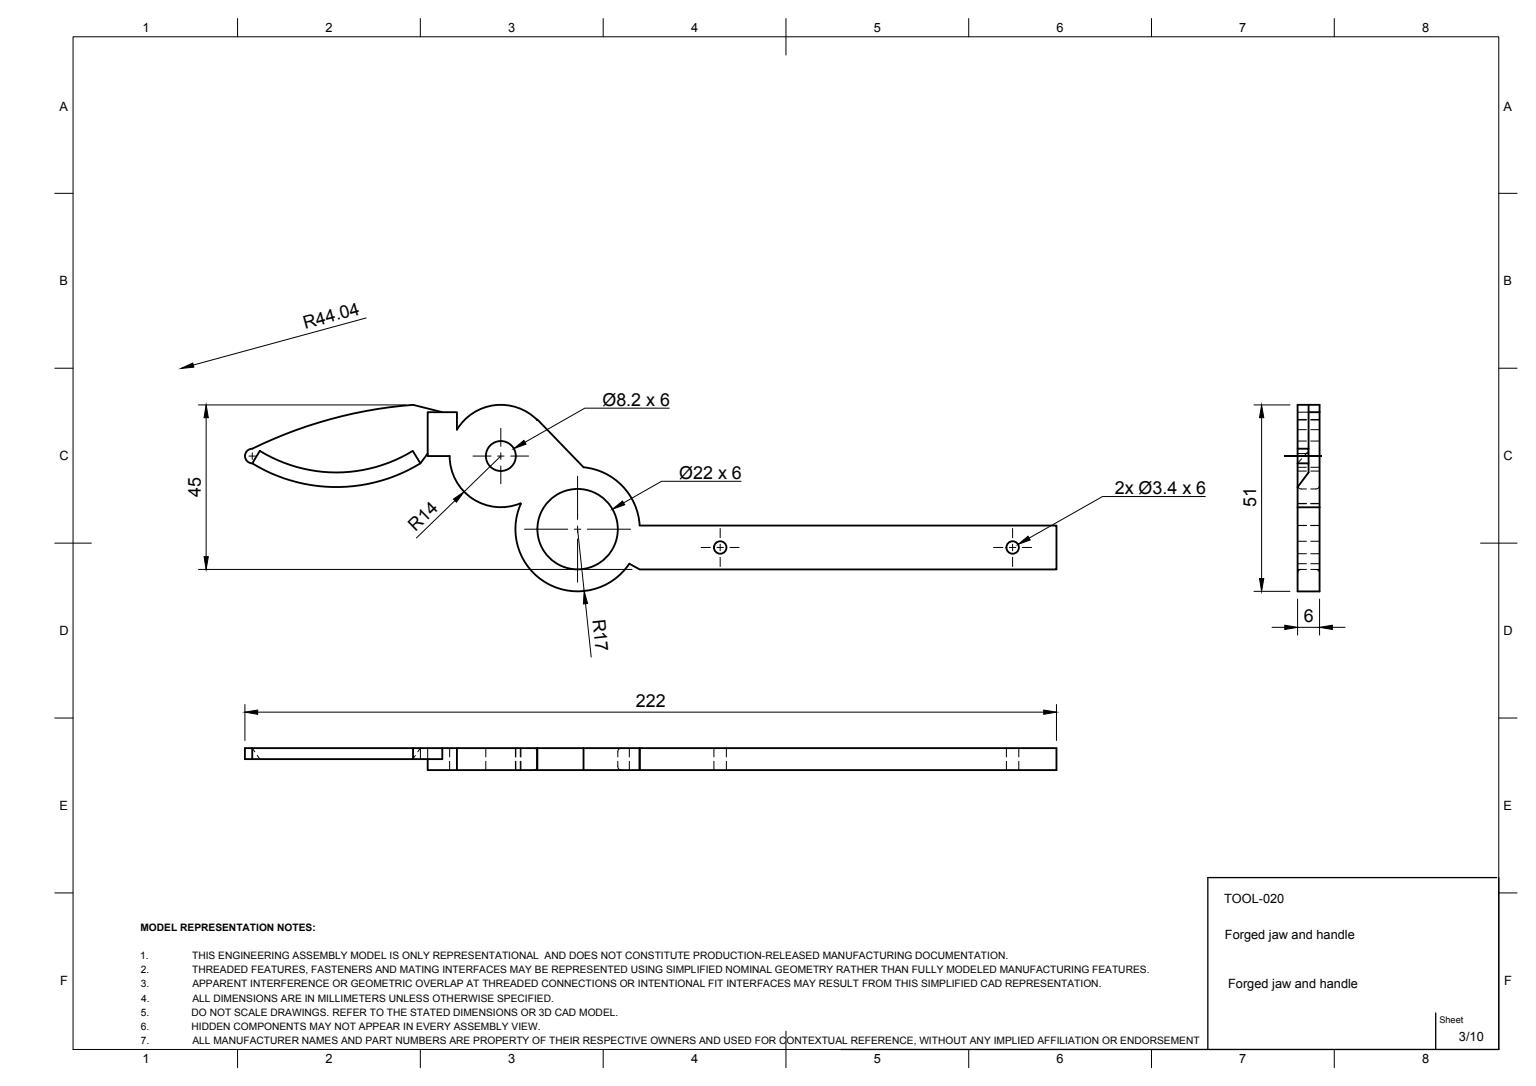
ISO-10303-21;
HEADER;
/* Generated by software containing ST-Developer
 * from STEP Tools, Inc. (www.steptools.com) 
 */

FILE_DESCRIPTION(
/* description */ (''),
/* implementation_level */ '2;1');

FILE_NAME(
/* name */ 'Forged jaw and handle.step',
/* time_stamp */ '2026-11-10T09:09:39-08:00',
/* author */ (''),
/* organization */ (''),
/* preprocessor_version */ 'ST-DEVELOPER v20.2',
/* originating_system */ 'Autodesk Translation Framework v15.17.0.0',
/* authorisation */ '');

FILE_SCHEMA (('AUTOMOTIVE_DESIGN { 1 0 10303 214 3 1 1 }'));
ENDSEC;

DATA;
#10=MECHANICAL_DESIGN_GEOMETRIC_PRESENTATION_REPRESENTATION('',(#555),#18353);
#537=SHAPE_REPRESENTATION_RELATIONSHIP('SRR','None',#18397,#546);
#546=ADVANCED_BREP_SHAPE_REPRESENTATION('',(#564),#18343);
#555=STYLED_ITEM('',(#18456),#564);
#564=MANIFOLD_SOLID_BREP('Body1',#6486);
#573=TOROIDAL_SURFACE('',#6634,1.2,0.1);
#574=TOROIDAL_SURFACE('',#6644,1.2,0.1);
#575=FACE_BOUND('',#1173,.T.);
#576=FACE_BOUND('',#1174,.T.);
#577=FACE_BOUND('',#1175,.T.);
#578=FACE_BOUND('',#1176,.T.);
#579=FACE_BOUND('',#1180,.T.);
#580=FACE_BOUND('',#1181,.T.);
#581=FACE_BOUND('',#1182,.T.);
#582=FACE_BOUND('',#1183,.T.);
#638=CONICAL_SURFACE('',#6607,4.2044765934785,0.927295218001611);
#640=PLANE('',#6606);
#641=PLANE('',#6610);
#642=PLANE('',#6611);
#643=PLANE('',#6612);
#644=PLANE('',#6619);
#645=PLANE('',#6620);
#646=PLANE('',#6621);
#647=PLANE('',#6622);
#648=PLANE('',#6623);
#649=PLANE('',#6630);
#650=PLANE('',#6641);
#651=PLANE('',#6648);
#652=PLANE('',#6649);
#653=PLANE('',#6650);
#654=PLANE('',#6651);
#655=PLANE('',#6652);
#656=PLANE('',#6653);
#657=PLANE('',#6654);
#658=PLANE('',#6655);
#782=FACE_OUTER_BOUND('',#1155,.T.);
#783=FACE_OUTER_BOUND('',#1156,.T.);
#784=FACE_OUTER_BOUND('',#1157,.T.);
#785=FACE_OUTER_BOUND('',#1158,.T.);
#786=FACE_OUTER_BOUND('',#1159,.T.);
#787=FACE_OUTER_BOUND('',#1160,.T.);
#788=FACE_OUTER_BOUND('',#1161,.T.);
#789=FACE_OUTER_BOUND('',#1162,.T.);
#790=FACE_OUTER_BOUND('',#1163,.T.);
#791=FACE_OUTER_BOUND('',#1164,.T.);
#792=FACE_OUTER_BOUND('',#1165,.T.);
#793=FACE_OUTER_BOUND('',#1166,.T.);
#794=FACE_OUTER_BOUND('',#1167,.T.);
#795=FACE_OUTER_BOUND('',#1168,.T.);
#796=FACE_OUTER_BOUND('',#1169,.T.);
#797=FACE_OUTER_BOUND('',#1170,.T.);
#798=FACE_OUTER_BOUND('',#1171,.T.);
#799=FACE_OUTER_BOUND('',#1172,.T.);
#800=FACE_OUTER_BOUND('',#1177,.T.);
#801=FACE_OUTER_BOUND('',#1178,.T.);
#802=FACE_OUTER_BOUND('',#1179,.T.);
#803=FACE_OUTER_BOUND('',#1184,.T.);
#804=FACE_OUTER_BOUND('',#1185,.T.);
#805=FACE_OUTER_BOUND('',#1186,.T.);
#806=FACE_OUTER_BOUND('',#1187,.T.);
#807=FACE_OUTER_BOUND('',#1188,.T.);
#808=FACE_OUTER_BOUND('',#1189,.T.);
#809=FACE_OUTER_BOUND('',#1190,.T.);
#810=FACE_OUTER_BOUND('',#1191,.T.);
#811=FACE_OUTER_BOUND('',#1192,.T.);
#812=FACE_OUTER_BOUND('',#1193,.T.);
#813=FACE_OUTER_BOUND('',#1194,.T.);
#1155=EDGE_LOOP('',(#4108,#4109,#4110,#4111));
#1156=EDGE_LOOP('',(#4112,#4113,#4114,#4115));
#1157=EDGE_LOOP('',(#4116,#4117,#4118,#4119));
#1158=EDGE_LOOP('',(#4120,#4121,#4122));
#1159=EDGE_LOOP('',(#4123,#4124,#4125,#4126));
#1160=EDGE_LOOP('',(#4127,#4128,#4129));
#1161=EDGE_LOOP('',(#4130,#4131,#4132,#4133));
#1162=EDGE_LOOP('',(#4134,#4135,#4136,#4137));
#1163=EDGE_LOOP('',(#4138,#4139,#4140,#4141));
#1164=EDGE_LOOP('',(#4142,#4143,#4144,#4145));
#1165=EDGE_LOOP('',(#4146,#4147,#4148,#4149,#4150,#4151,#4152,#4153,#4154));
#1166=EDGE_LOOP('',(#4155,#4156,#4157,#4158,#4159,#4160));
#1167=EDGE_LOOP('',(#4161,#4162,#4163,#4164,#4165,#4166));
#1168=EDGE_LOOP('',(#4167,#4168,#4169,#4170));
#1169=EDGE_LOOP('',(#4171,#4172,#4173,#4174));
#1170=EDGE_LOOP('',(#4175,#4176,#4177,#4178));
#1171=EDGE_LOOP('',(#4179,#4180,#4181,#4182));
#1172=EDGE_LOOP('',(#4183,#4184,#4185,#4186,#4187,#4188,#4189,#4190,#4191,
#4192,#4193,#4194,#4195,#4196,#4197,#4198));
#1173=EDGE_LOOP('',(#4199));
#1174=EDGE_LOOP('',(#4200));
#1175=EDGE_LOOP('',(#4201));
#1176=EDGE_LOOP('',(#4202));
#1177=EDGE_LOOP('',(#4203,#4204,#4205,#4206));
#1178=EDGE_LOOP('',(#4207,#4208,#4209,#4210,#4211));
#1179=EDGE_LOOP('',(#4212,#4213,#4214,#4215,#4216,#4217,#4218,#4219,#4220,
#4221,#4222,#4223,#4224,#4225,#4226,#4227,#4228,#4229,#4230,#4231,#4232));
#1180=EDGE_LOOP('',(#4233));
#1181=EDGE_LOOP('',(#4234));
#1182=EDGE_LOOP('',(#4235));
#1183=EDGE_LOOP('',(#4236));
#1184=EDGE_LOOP('',(#4237,#4238,#4239,#4240,#4241));
#1185=EDGE_LOOP('',(#4242,#4243,#4244,#4245));
#1186=EDGE_LOOP('',(#4246,#4247,#4248,#4249));
#1187=EDGE_LOOP('',(#4250,#4251,#4252,#4253));
#1188=EDGE_LOOP('',(#4254,#4255,#4256,#4257));
#1189=EDGE_LOOP('',(#4258,#4259,#4260,#4261));
#1190=EDGE_LOOP('',(#4262,#4263,#4264,#4265));
#1191=EDGE_LOOP('',(#4266,#4267,#4268,#4269));
#1192=EDGE_LOOP('',(#4270,#4271,#4272,#4273));
#1193=EDGE_LOOP('',(#4274,#4275,#4276,#4277));
#1194=EDGE_LOOP('',(#4278,#4279,#4280,#4281));
#1591=LINE('',#8466,#1995);
#1592=LINE('',#8472,#1996);
#1593=LINE('',#8478,#1997);
#1594=LINE('',#8483,#1998);
#1595=LINE('',#8485,#1999);
#1596=LINE('',#8486,#2000);
#1597=LINE('',#8490,#2001);
#1598=LINE('',#8495,#2002);
#1599=LINE('',#8496,#2003);
#1600=LINE('',#8500,#2004);
#1601=LINE('',#8501,#2005);
#1602=LINE('',#8502,#2006);
#1603=LINE('',#8506,#2007);
#1604=LINE('',#8508,#2008);
#1605=LINE('',#8510,#2009);
#1606=LINE('',#8511,#2010);
#1607=LINE('',#8517,#2011);
#1608=LINE('',#8523,#2012);
#1609=LINE('',#8524,#2013);
#1610=LINE('',#8527,#2014);
#1611=LINE('',#8529,#2015);
#1612=LINE('',#8531,#2016);
#1613=LINE('',#8532,#2017);
#1614=LINE('',#8535,#2018);
#1615=LINE('',#8537,#2019);
#1616=LINE('',#8538,#2020);
#1617=LINE('',#8542,#2021);
#1618=LINE('',#8543,#2022);
#1619=LINE('',#8544,#2023);
#1620=LINE('',#8548,#2024);
#1621=LINE('',#8549,#2025);
#1622=LINE('',#8550,#2026);
#1623=LINE('',#8555,#2027);
#1624=LINE('',#8561,#2028);
#1625=LINE('',#8565,#2029);
#1626=LINE('',#8569,#2030);
#1627=LINE('',#8571,#2031);
#1628=LINE('',#8573,#2032);
#1629=LINE('',#8575,#2033);
#1630=LINE('',#8577,#2034);
#1631=LINE('',#8581,#2035);
#1632=LINE('',#8582,#2036);
#1633=LINE('',#8596,#2037);
#1634=LINE('',#8599,#2038);
#1635=LINE('',#8601,#2039);
#1636=LINE('',#8605,#2040);
#1637=LINE('',#8607,#2041);
#1638=LINE('',#8609,#2042);
#1639=LINE('',#8611,#2043);
#1640=LINE('',#8613,#2044);
#1641=LINE('',#8616,#2045);
#1642=LINE('',#8620,#2046);
#1643=LINE('',#8621,#2047);
#1644=LINE('',#8623,#2048);
#1645=LINE('',#8624,#2049);
#1646=LINE('',#8626,#2050);
#1647=LINE('',#8628,#2051);
#1648=LINE('',#8631,#2052);
#1649=LINE('',#8634,#2053);
#1650=LINE('',#8636,#2054);
#1995=VECTOR('',#7090,0.17);
#1996=VECTOR('',#7097,0.17);
#1997=VECTOR('',#7104,0.41);
#1998=VECTOR('',#7109,1.);
#1999=VECTOR('',#7110,1.);
#2000=VECTOR('',#7111,1.);
#2001=VECTOR('',#7114,1.);
#2002=VECTOR('',#7121,1.);
#2003=VECTOR('',#7122,1.);
#2004=VECTOR('',#7125,1.);
#2005=VECTOR('',#7126,1.);
#2006=VECTOR('',#7127,1.);
#2007=VECTOR('',#7130,1.);
#2008=VECTOR('',#7131,1.);
#2009=VECTOR('',#7132,1.);
#2010=VECTOR('',#7133,1.);
#2011=VECTOR('',#7140,1.);
#2012=VECTOR('',#7149,1.);
#2013=VECTOR('',#7150,1.);
#2014=VECTOR('',#7153,1.);
#2015=VECTOR('',#7154,1.);
#2016=VECTOR('',#7155,1.);
#2017=VECTOR('',#7156,1.);
#2018=VECTOR('',#7159,1.);
#2019=VECTOR('',#7160,1.);
#2020=VECTOR('',#7161,1.);
#2021=VECTOR('',#7164,1.);
#2022=VECTOR('',#7165,1.);
#2023=VECTOR('',#7166,1.);
#2024=VECTOR('',#7169,1.);
#2025=VECTOR('',#7170,1.);
#2026=VECTOR('',#7171,1.);
#2027=VECTOR('',#7176,1.);
#2028=VECTOR('',#7183,1.);
#2029=VECTOR('',#7188,1.);
#2030=VECTOR('',#7191,1.);
#2031=VECTOR('',#7192,1.);
#2032=VECTOR('',#7193,1.);
#2033=VECTOR('',#7194,1.);
#2034=VECTOR('',#7195,1.);
#2035=VECTOR('',#7198,1.);
#2036=VECTOR('',#7199,1.);
#2037=VECTOR('',#7216,1.1);
#2038=VECTOR('',#7219,1.);
#2039=VECTOR('',#7220,1.);
#2040=VECTOR('',#7223,1.);
#2041=VECTOR('',#7224,1.);
#2042=VECTOR('',#7225,1.);
#2043=VECTOR('',#7226,1.);
#2044=VECTOR('',#7227,1.);
#2045=VECTOR('',#7230,1.);
#2046=VECTOR('',#7237,1.);
#2047=VECTOR('',#7238,1.);
#2048=VECTOR('',#7241,1.);
#2049=VECTOR('',#7242,1.);
#2050=VECTOR('',#7245,1.);
#2051=VECTOR('',#7248,1.);
#2052=VECTOR('',#7253,1.);
#2053=VECTOR('',#7258,1.);
#2054=VECTOR('',#7261,1.);
#2399=CIRCLE('',#6598,0.17);
#2400=CIRCLE('',#6599,0.17);
#2401=CIRCLE('',#6601,0.17);
#2402=CIRCLE('',#6602,0.17);
#2403=CIRCLE('',#6604,0.41);
#2404=CIRCLE('',#6605,0.41);
#2405=CIRCLE('',#6608,4.4044765934785);
#2406=CIRCLE('',#6609,4.0044765934785);
#2407=CIRCLE('',#6614,0.2);
#2408=CIRCLE('',#6615,0.2);
#2409=CIRCLE('',#6617,12.0894198846614);
#2410=CIRCLE('',#6618,12.0894198846614);
#2411=CIRCLE('',#6625,1.4);
#2412=CIRCLE('',#6626,1.4);
#2413=CIRCLE('',#6628,1.4);
#2414=CIRCLE('',#6629,1.4);
#2415=CIRCLE('',#6631,1.7);
#2416=CIRCLE('',#6632,1.7);
#2417=CIRCLE('',#6633,1.2);
#2418=CIRCLE('',#6635,1.2);
#2419=CIRCLE('',#6636,0.1);
#2420=CIRCLE('',#6637,1.1);
#2421=CIRCLE('',#6639,1.1);
#2422=CIRCLE('',#6640,1.1);
#2423=CIRCLE('',#6642,1.7);
#2424=CIRCLE('',#6643,1.7);
#2425=CIRCLE('',#6645,0.1);
#2566=VERTEX_POINT('',#8463);
#2567=VERTEX_POINT('',#8465);
#2568=VERTEX_POINT('',#8469);
#2569=VERTEX_POINT('',#8471);
#2570=VERTEX_POINT('',#8475);
#2571=VERTEX_POINT('',#8477);
#2572=VERTEX_POINT('',#8481);
#2573=VERTEX_POINT('',#8482);
#2574=VERTEX_POINT('',#8484);
#2575=VERTEX_POINT('',#8488);
#2576=VERTEX_POINT('',#8489);
#2577=VERTEX_POINT('',#8494);
#2578=VERTEX_POINT('',#8498);
#2579=VERTEX_POINT('',#8499);
#2580=VERTEX_POINT('',#8504);
#2581=VERTEX_POINT('',#8505);
#2582=VERTEX_POINT('',#8507);
#2583=VERTEX_POINT('',#8509);
#2584=VERTEX_POINT('',#8513);
#2585=VERTEX_POINT('',#8515);
#2586=VERTEX_POINT('',#8522);
#2587=VERTEX_POINT('',#8526);
#2588=VERTEX_POINT('',#8528);
#2589=VERTEX_POINT('',#8530);
#2590=VERTEX_POINT('',#8534);
#2591=VERTEX_POINT('',#8536);
#2592=VERTEX_POINT('',#8540);
#2593=VERTEX_POINT('',#8541);
#2594=VERTEX_POINT('',#8546);
#2595=VERTEX_POINT('',#8547);
#2596=VERTEX_POINT('',#8552);
#2597=VERTEX_POINT('',#8554);
#2598=VERTEX_POINT('',#8558);
#2599=VERTEX_POINT('',#8560);
#2600=VERTEX_POINT('',#8564);
#2601=VERTEX_POINT('',#8566);
#2602=VERTEX_POINT('',#8568);
#2603=VERTEX_POINT('',#8570);
#2604=VERTEX_POINT('',#8572);
#2605=VERTEX_POINT('',#8574);
#2606=VERTEX_POINT('',#8576);
#2607=VERTEX_POINT('',#8578);
#2608=VERTEX_POINT('',#8580);
#2609=VERTEX_POINT('',#8583);
#2610=VERTEX_POINT('',#8586);
#2611=VERTEX_POINT('',#8588);
#2612=VERTEX_POINT('',#8592);
#2613=VERTEX_POINT('',#8593);
#2614=VERTEX_POINT('',#8598);
#2615=VERTEX_POINT('',#8600);
#2616=VERTEX_POINT('',#8602);
#2617=VERTEX_POINT('',#8604);
#2618=VERTEX_POINT('',#8606);
#2619=VERTEX_POINT('',#8608);
#2620=VERTEX_POINT('',#8610);
#2621=VERTEX_POINT('',#8612);
#2622=VERTEX_POINT('',#8614);
#3171=EDGE_CURVE('',#2566,#2566,#2399,.T.);
#3172=EDGE_CURVE('',#2566,#2567,#1591,.T.);
#3173=EDGE_CURVE('',#2567,#2567,#2400,.T.);
#3174=EDGE_CURVE('',#2568,#2568,#2401,.T.);
#3175=EDGE_CURVE('',#2568,#2569,#1592,.T.);
#3176=EDGE_CURVE('',#2569,#2569,#2402,.T.);
#3177=EDGE_CURVE('',#2570,#2570,#2403,.T.);
#3178=EDGE_CURVE('',#2570,#2571,#1593,.T.);
#3179=EDGE_CURVE('',#2571,#2571,#2404,.T.);
#3180=EDGE_CURVE('',#2572,#2573,#1594,.T.);
#3181=EDGE_CURVE('',#2574,#2572,#1595,.T.);
#3182=EDGE_CURVE('',#2574,#2573,#1596,.T.);
#3183=EDGE_CURVE('',#2575,#2576,#1597,.T.);
#3184=EDGE_CURVE('',#2575,#2574,#2405,.T.);
#3185=EDGE_CURVE('',#2576,#2572,#2406,.T.);
#3186=EDGE_CURVE('',#2577,#2576,#1598,.T.);
#3187=EDGE_CURVE('',#2575,#2577,#1599,.T.);
#3188=EDGE_CURVE('',#2578,#2579,#1600,.T.);
#3189=EDGE_CURVE('',#2573,#2578,#1601,.T.);
#3190=EDGE_CURVE('',#2579,#2574,#1602,.T.);
#3191=EDGE_CURVE('',#2580,#2581,#1603,.T.);
#3192=EDGE_CURVE('',#2580,#2582,#1604,.T.);
#3193=EDGE_CURVE('',#2583,#2582,#1605,.T.);
#3194=EDGE_CURVE('',#2581,#2583,#1606,.T.);
#3195=EDGE_CURVE('',#2584,#2575,#2407,.T.);
#3196=EDGE_CURVE('',#2585,#2577,#2408,.T.);
#3197=EDGE_CURVE('',#2584,#2585,#1607,.T.);
#3198=EDGE_CURVE('',#2580,#2584,#2409,.T.);
#3199=EDGE_CURVE('',#2582,#2585,#2410,.T.);
#3200=EDGE_CURVE('',#2586,#2578,#1608,.T.);
#3201=EDGE_CURVE('',#2583,#2586,#1609,.T.);
#3202=EDGE_CURVE('',#2586,#2587,#1610,.T.);
#3203=EDGE_CURVE('',#2588,#2587,#1611,.T.);
#3204=EDGE_CURVE('',#2589,#2588,#1612,.T.);
#3205=EDGE_CURVE('',#2581,#2589,#1613,.T.);
#3206=EDGE_CURVE('',#2590,#2579,#1614,.T.);
#3207=EDGE_CURVE('',#2590,#2591,#1615,.T.);
#3208=EDGE_CURVE('',#2587,#2591,#1616,.T.);
#3209=EDGE_CURVE('',#2592,#2593,#1617,.T.);
#3210=EDGE_CURVE('',#2591,#2592,#1618,.T.);
#3211=EDGE_CURVE('',#2593,#2590,#1619,.T.);
#3212=EDGE_CURVE('',#2594,#2595,#1620,.T.);
#3213=EDGE_CURVE('',#2589,#2594,#1621,.T.);
#3214=EDGE_CURVE('',#2595,#2588,#1622,.T.);
#3215=EDGE_CURVE('',#2593,#2596,#2411,.T.);
#3216=EDGE_CURVE('',#2596,#2597,#1623,.T.);
#3217=EDGE_CURVE('',#2592,#2597,#2412,.T.);
#3218=EDGE_CURVE('',#2598,#2595,#2413,.T.);
#3219=EDGE_CURVE('',#2598,#2599,#1624,.T.);
#3220=EDGE_CURVE('',#2599,#2594,#2414,.T.);
#3221=EDGE_CURVE('',#2597,#2600,#1625,.T.);
#3222=EDGE_CURVE('',#2600,#2601,#2415,.T.);
#3223=EDGE_CURVE('',#2601,#2602,#1626,.T.);
#3224=EDGE_CURVE('',#2602,#2603,#1627,.T.);
#3225=EDGE_CURVE('',#2603,#2604,#1628,.T.);
#3226=EDGE_CURVE('',#2604,#2605,#1629,.T.);
#3227=EDGE_CURVE('',#2605,#2606,#1630,.T.);
#3228=EDGE_CURVE('',#2606,#2607,#2416,.T.);
#3229=EDGE_CURVE('',#2607,#2608,#1631,.T.);
#3230=EDGE_CURVE('',#2608,#2598,#1632,.T.);
#3231=EDGE_CURVE('',#2609,#2609,#2417,.T.);
#3232=EDGE_CURVE('',#2610,#2610,#2418,.T.);
#3233=EDGE_CURVE('',#2610,#2611,#2419,.T.);
#3234=EDGE_CURVE('',#2611,#2611,#2420,.T.);
#3235=EDGE_CURVE('',#2612,#2613,#2421,.T.);
#3236=EDGE_CURVE('',#2613,#2612,#2422,.T.);
#3237=EDGE_CURVE('',#2613,#2611,#1633,.T.);
#3238=EDGE_CURVE('',#2614,#2599,#1634,.T.);
#3239=EDGE_CURVE('',#2615,#2614,#1635,.T.);
#3240=EDGE_CURVE('',#2616,#2615,#2423,.T.);
#3241=EDGE_CURVE('',#2617,#2616,#1636,.T.);
#3242=EDGE_CURVE('',#2618,#2617,#1637,.T.);
#3243=EDGE_CURVE('',#2619,#2618,#1638,.T.);
#3244=EDGE_CURVE('',#2620,#2619,#1639,.T.);
#3245=EDGE_CURVE('',#2621,#2620,#1640,.T.);
#3246=EDGE_CURVE('',#2622,#2621,#2424,.T.);
#3247=EDGE_CURVE('',#2596,#2622,#1641,.T.);
#3248=EDGE_CURVE('',#2609,#2612,#2425,.T.);
#3249=EDGE_CURVE('',#2607,#2615,#1642,.T.);
#3250=EDGE_CURVE('',#2616,#2606,#1643,.T.);
#3251=EDGE_CURVE('',#2622,#2600,#1644,.T.);
#3252=EDGE_CURVE('',#2601,#2621,#1645,.T.);
#3253=EDGE_CURVE('',#2620,#2602,#1646,.T.);
#3254=EDGE_CURVE('',#2617,#2605,#1647,.T.);
#3255=EDGE_CURVE('',#2614,#2608,#1648,.T.);
#3256=EDGE_CURVE('',#2618,#2604,#1649,.T.);
#3257=EDGE_CURVE('',#2619,#2603,#1650,.T.);
#4108=ORIENTED_EDGE('',*,*,#3171,.F.);
#4109=ORIENTED_EDGE('',*,*,#3172,.T.);
#4110=ORIENTED_EDGE('',*,*,#3173,.F.);
#4111=ORIENTED_EDGE('',*,*,#3172,.F.);
#4112=ORIENTED_EDGE('',*,*,#3174,.F.);
#4113=ORIENTED_EDGE('',*,*,#3175,.T.);
#4114=ORIENTED_EDGE('',*,*,#3176,.F.);
#4115=ORIENTED_EDGE('',*,*,#3175,.F.);
#4116=ORIENTED_EDGE('',*,*,#3177,.F.);
#4117=ORIENTED_EDGE('',*,*,#3178,.T.);
#4118=ORIENTED_EDGE('',*,*,#3179,.F.);
#4119=ORIENTED_EDGE('',*,*,#3178,.F.);
#4120=ORIENTED_EDGE('',*,*,#3180,.F.);
#4121=ORIENTED_EDGE('',*,*,#3181,.F.);
#4122=ORIENTED_EDGE('',*,*,#3182,.T.);
#4123=ORIENTED_EDGE('',*,*,#3183,.F.);
#4124=ORIENTED_EDGE('',*,*,#3184,.T.);
#4125=ORIENTED_EDGE('',*,*,#3181,.T.);
#4126=ORIENTED_EDGE('',*,*,#3185,.F.);
#4127=ORIENTED_EDGE('',*,*,#3186,.F.);
#4128=ORIENTED_EDGE('',*,*,#3187,.F.);
#4129=ORIENTED_EDGE('',*,*,#3183,.T.);
#4130=ORIENTED_EDGE('',*,*,#3188,.F.);
#4131=ORIENTED_EDGE('',*,*,#3189,.F.);
#4132=ORIENTED_EDGE('',*,*,#3182,.F.);
#4133=ORIENTED_EDGE('',*,*,#3190,.F.);
#4134=ORIENTED_EDGE('',*,*,#3191,.F.);
#4135=ORIENTED_EDGE('',*,*,#3192,.T.);
#4136=ORIENTED_EDGE('',*,*,#3193,.F.);
#4137=ORIENTED_EDGE('',*,*,#3194,.F.);
#4138=ORIENTED_EDGE('',*,*,#3195,.T.);
#4139=ORIENTED_EDGE('',*,*,#3187,.T.);
#4140=ORIENTED_EDGE('',*,*,#3196,.F.);
#4141=ORIENTED_EDGE('',*,*,#3197,.F.);
#4142=ORIENTED_EDGE('',*,*,#3198,.T.);
#4143=ORIENTED_EDGE('',*,*,#3197,.T.);
#4144=ORIENTED_EDGE('',*,*,#3199,.F.);
#4145=ORIENTED_EDGE('',*,*,#3192,.F.);
#4146=ORIENTED_EDGE('',*,*,#3180,.T.);
#4147=ORIENTED_EDGE('',*,*,#3189,.T.);
#4148=ORIENTED_EDGE('',*,*,#3200,.F.);
#4149=ORIENTED_EDGE('',*,*,#3201,.F.);
#4150=ORIENTED_EDGE('',*,*,#3193,.T.);
#4151=ORIENTED_EDGE('',*,*,#3199,.T.);
#4152=ORIENTED_EDGE('',*,*,#3196,.T.);
#4153=ORIENTED_EDGE('',*,*,#3186,.T.);
#4154=ORIENTED_EDGE('',*,*,#3185,.T.);
#4155=ORIENTED_EDGE('',*,*,#3194,.T.);
#4156=ORIENTED_EDGE('',*,*,#3201,.T.);
#4157=ORIENTED_EDGE('',*,*,#3202,.T.);
#4158=ORIENTED_EDGE('',*,*,#3203,.F.);
#4159=ORIENTED_EDGE('',*,*,#3204,.F.);
#4160=ORIENTED_EDGE('',*,*,#3205,.F.);
#4161=ORIENTED_EDGE('',*,*,#3200,.T.);
#4162=ORIENTED_EDGE('',*,*,#3188,.T.);
#4163=ORIENTED_EDGE('',*,*,#3206,.F.);
#4164=ORIENTED_EDGE('',*,*,#3207,.T.);
#4165=ORIENTED_EDGE('',*,*,#3208,.F.);
#4166=ORIENTED_EDGE('',*,*,#3202,.F.);
#4167=ORIENTED_EDGE('',*,*,#3209,.F.);
#4168=ORIENTED_EDGE('',*,*,#3210,.F.);
#4169=ORIENTED_EDGE('',*,*,#3207,.F.);
#4170=ORIENTED_EDGE('',*,*,#3211,.F.);
#4171=ORIENTED_EDGE('',*,*,#3212,.F.);
#4172=ORIENTED_EDGE('',*,*,#3213,.F.);
#4173=ORIENTED_EDGE('',*,*,#3204,.T.);
#4174=ORIENTED_EDGE('',*,*,#3214,.F.);
#4175=ORIENTED_EDGE('',*,*,#3209,.T.);
#4176=ORIENTED_EDGE('',*,*,#3215,.T.);
#4177=ORIENTED_EDGE('',*,*,#3216,.T.);
#4178=ORIENTED_EDGE('',*,*,#3217,.F.);
#4179=ORIENTED_EDGE('',*,*,#3212,.T.);
#4180=ORIENTED_EDGE('',*,*,#3218,.F.);
#4181=ORIENTED_EDGE('',*,*,#3219,.T.);
#4182=ORIENTED_EDGE('',*,*,#3220,.T.);
#4183=ORIENTED_EDGE('',*,*,#3217,.T.);
#4184=ORIENTED_EDGE('',*,*,#3221,.T.);
#4185=ORIENTED_EDGE('',*,*,#3222,.T.);
#4186=ORIENTED_EDGE('',*,*,#3223,.T.);
#4187=ORIENTED_EDGE('',*,*,#3224,.T.);
#4188=ORIENTED_EDGE('',*,*,#3225,.T.);
#4189=ORIENTED_EDGE('',*,*,#3226,.T.);
#4190=ORIENTED_EDGE('',*,*,#3227,.T.);
#4191=ORIENTED_EDGE('',*,*,#3228,.T.);
#4192=ORIENTED_EDGE('',*,*,#3229,.T.);
#4193=ORIENTED_EDGE('',*,*,#3230,.T.);
#4194=ORIENTED_EDGE('',*,*,#3218,.T.);
#4195=ORIENTED_EDGE('',*,*,#3214,.T.);
#4196=ORIENTED_EDGE('',*,*,#3203,.T.);
#4197=ORIENTED_EDGE('',*,*,#3208,.T.);
#4198=ORIENTED_EDGE('',*,*,#3210,.T.);
#4199=ORIENTED_EDGE('',*,*,#3171,.T.);
#4200=ORIENTED_EDGE('',*,*,#3174,.T.);
#4201=ORIENTED_EDGE('',*,*,#3177,.T.);
#4202=ORIENTED_EDGE('',*,*,#3231,.F.);
#4203=ORIENTED_EDGE('',*,*,#3232,.T.);
#4204=ORIENTED_EDGE('',*,*,#3233,.T.);
#4205=ORIENTED_EDGE('',*,*,#3234,.T.);
#4206=ORIENTED_EDGE('',*,*,#3233,.F.);
#4207=ORIENTED_EDGE('',*,*,#3235,.F.);
#4208=ORIENTED_EDGE('',*,*,#3236,.F.);
#4209=ORIENTED_EDGE('',*,*,#3237,.T.);
#4210=ORIENTED_EDGE('',*,*,#3234,.F.);
#4211=ORIENTED_EDGE('',*,*,#3237,.F.);
#4212=ORIENTED_EDGE('',*,*,#3205,.T.);
#4213=ORIENTED_EDGE('',*,*,#3213,.T.);
#4214=ORIENTED_EDGE('',*,*,#3220,.F.);
#4215=ORIENTED_EDGE('',*,*,#3238,.F.);
#4216=ORIENTED_EDGE('',*,*,#3239,.F.);
#4217=ORIENTED_EDGE('',*,*,#3240,.F.);
#4218=ORIENTED_EDGE('',*,*,#3241,.F.);
#4219=ORIENTED_EDGE('',*,*,#3242,.F.);
#4220=ORIENTED_EDGE('',*,*,#3243,.F.);
#4221=ORIENTED_EDGE('',*,*,#3244,.F.);
#4222=ORIENTED_EDGE('',*,*,#3245,.F.);
#4223=ORIENTED_EDGE('',*,*,#3246,.F.);
#4224=ORIENTED_EDGE('',*,*,#3247,.F.);
#4225=ORIENTED_EDGE('',*,*,#3215,.F.);
#4226=ORIENTED_EDGE('',*,*,#3211,.T.);
#4227=ORIENTED_EDGE('',*,*,#3206,.T.);
#4228=ORIENTED_EDGE('',*,*,#3190,.T.);
#4229=ORIENTED_EDGE('',*,*,#3184,.F.);
#4230=ORIENTED_EDGE('',*,*,#3195,.F.);
#4231=ORIENTED_EDGE('',*,*,#3198,.F.);
#4232=ORIENTED_EDGE('',*,*,#3191,.T.);
#4233=ORIENTED_EDGE('',*,*,#3173,.T.);
#4234=ORIENTED_EDGE('',*,*,#3176,.T.);
#4235=ORIENTED_EDGE('',*,*,#3179,.T.);
#4236=ORIENTED_EDGE('',*,*,#3232,.F.);
#4237=ORIENTED_EDGE('',*,*,#3231,.T.);
#4238=ORIENTED_EDGE('',*,*,#3248,.T.);
#4239=ORIENTED_EDGE('',*,*,#3235,.T.);
#4240=ORIENTED_EDGE('',*,*,#3236,.T.);
#4241=ORIENTED_EDGE('',*,*,#3248,.F.);
#4242=ORIENTED_EDGE('',*,*,#3249,.F.);
#4243=ORIENTED_EDGE('',*,*,#3228,.F.);
#4244=ORIENTED_EDGE('',*,*,#3250,.F.);
#4245=ORIENTED_EDGE('',*,*,#3240,.T.);
#4246=ORIENTED_EDGE('',*,*,#3251,.F.);
#4247=ORIENTED_EDGE('',*,*,#3246,.T.);
#4248=ORIENTED_EDGE('',*,*,#3252,.F.);
#4249=ORIENTED_EDGE('',*,*,#3222,.F.);
#4250=ORIENTED_EDGE('',*,*,#3252,.T.);
#4251=ORIENTED_EDGE('',*,*,#3245,.T.);
#4252=ORIENTED_EDGE('',*,*,#3253,.T.);
#4253=ORIENTED_EDGE('',*,*,#3223,.F.);
#4254=ORIENTED_EDGE('',*,*,#3250,.T.);
#4255=ORIENTED_EDGE('',*,*,#3227,.F.);
#4256=ORIENTED_EDGE('',*,*,#3254,.F.);
#4257=ORIENTED_EDGE('',*,*,#3241,.T.);
#4258=ORIENTED_EDGE('',*,*,#3251,.T.);
#4259=ORIENTED_EDGE('',*,*,#3221,.F.);
#4260=ORIENTED_EDGE('',*,*,#3216,.F.);
#4261=ORIENTED_EDGE('',*,*,#3247,.T.);
#4262=ORIENTED_EDGE('',*,*,#3219,.F.);
#4263=ORIENTED_EDGE('',*,*,#3230,.F.);
#4264=ORIENTED_EDGE('',*,*,#3255,.F.);
#4265=ORIENTED_EDGE('',*,*,#3238,.T.);
#4266=ORIENTED_EDGE('',*,*,#3249,.T.);
#4267=ORIENTED_EDGE('',*,*,#3239,.T.);
#4268=ORIENTED_EDGE('',*,*,#3255,.T.);
#4269=ORIENTED_EDGE('',*,*,#3229,.F.);
#4270=ORIENTED_EDGE('',*,*,#3242,.T.);
#4271=ORIENTED_EDGE('',*,*,#3254,.T.);
#4272=ORIENTED_EDGE('',*,*,#3226,.F.);
#4273=ORIENTED_EDGE('',*,*,#3256,.F.);
#4274=ORIENTED_EDGE('',*,*,#3243,.T.);
#4275=ORIENTED_EDGE('',*,*,#3256,.T.);
#4276=ORIENTED_EDGE('',*,*,#3225,.F.);
#4277=ORIENTED_EDGE('',*,*,#3257,.F.);
#4278=ORIENTED_EDGE('',*,*,#3244,.T.);
#4279=ORIENTED_EDGE('',*,*,#3257,.T.);
#4280=ORIENTED_EDGE('',*,*,#3224,.F.);
#4281=ORIENTED_EDGE('',*,*,#3253,.F.);
#5982=CYLINDRICAL_SURFACE('',#6597,0.17);
#5983=CYLINDRICAL_SURFACE('',#6600,0.17);
#5984=CYLINDRICAL_SURFACE('',#6603,0.41);
#5985=CYLINDRICAL_SURFACE('',#6613,0.2);
#5986=CYLINDRICAL_SURFACE('',#6616,12.0894198846614);
#5987=CYLINDRICAL_SURFACE('',#6624,1.4);
#5988=CYLINDRICAL_SURFACE('',#6627,1.4);
#5989=CYLINDRICAL_SURFACE('',#6638,1.1);
#5990=CYLINDRICAL_SURFACE('',#6646,1.7);
#5991=CYLINDRICAL_SURFACE('',#6647,1.7);
#6113=ADVANCED_FACE('',(#782),#5982,.F.);
#6114=ADVANCED_FACE('',(#783),#5983,.F.);
#6115=ADVANCED_FACE('',(#784),#5984,.F.);
#6116=ADVANCED_FACE('',(#785),#640,.F.);
#6117=ADVANCED_FACE('',(#786),#638,.T.);
#6118=ADVANCED_FACE('',(#787),#641,.T.);
#6119=ADVANCED_FACE('',(#788),#642,.T.);
#6120=ADVANCED_FACE('',(#789),#643,.T.);
#6121=ADVANCED_FACE('',(#790),#5985,.T.);
#6122=ADVANCED_FACE('',(#791),#5986,.T.);
#6123=ADVANCED_FACE('',(#792),#644,.T.);
#6124=ADVANCED_FACE('',(#793),#645,.T.);
#6125=ADVANCED_FACE('',(#794),#646,.T.);
#6126=ADVANCED_FACE('',(#795),#647,.T.);
#6127=ADVANCED_FACE('',(#796),#648,.T.);
#6128=ADVANCED_FACE('',(#797),#5987,.T.);
#6129=ADVANCED_FACE('',(#798),#5988,.T.);
#6130=ADVANCED_FACE('',(#799,#575,#576,#577,#578),#649,.T.);
#6131=ADVANCED_FACE('',(#800),#573,.T.);
#6132=ADVANCED_FACE('',(#801),#5989,.F.);
#6133=ADVANCED_FACE('',(#802,#579,#580,#581,#582),#650,.F.);
#6134=ADVANCED_FACE('',(#803),#574,.T.);
#6135=ADVANCED_FACE('',(#804),#5990,.T.);
#6136=ADVANCED_FACE('',(#805),#5991,.T.);
#6137=ADVANCED_FACE('',(#806),#651,.T.);
#6138=ADVANCED_FACE('',(#807),#652,.T.);
#6139=ADVANCED_FACE('',(#808),#653,.T.);
#6140=ADVANCED_FACE('',(#809),#654,.T.);
#6141=ADVANCED_FACE('',(#810),#655,.T.);
#6142=ADVANCED_FACE('',(#811),#656,.T.);
#6143=ADVANCED_FACE('',(#812),#657,.T.);
#6144=ADVANCED_FACE('',(#813),#658,.T.);
#6486=CLOSED_SHELL('',(#6113,#6114,#6115,#6116,#6117,#6118,#6119,#6120,
#6121,#6122,#6123,#6124,#6125,#6126,#6127,#6128,#6129,#6130,#6131,#6132,
#6133,#6134,#6135,#6136,#6137,#6138,#6139,#6140,#6141,#6142,#6143,#6144));
#6596=AXIS2_PLACEMENT_3D('',#8461,#7084,#7085);
#6597=AXIS2_PLACEMENT_3D('',#8462,#7086,#7087);
#6598=AXIS2_PLACEMENT_3D('',#8464,#7088,#7089);
#6599=AXIS2_PLACEMENT_3D('',#8467,#7091,#7092);
#6600=AXIS2_PLACEMENT_3D('',#8468,#7093,#7094);
#6601=AXIS2_PLACEMENT_3D('',#8470,#7095,#7096);
#6602=AXIS2_PLACEMENT_3D('',#8473,#7098,#7099);
#6603=AXIS2_PLACEMENT_3D('',#8474,#7100,#7101);
#6604=AXIS2_PLACEMENT_3D('',#8476,#7102,#7103);
#6605=AXIS2_PLACEMENT_3D('',#8479,#7105,#7106);
#6606=AXIS2_PLACEMENT_3D('',#8480,#7107,#7108);
#6607=AXIS2_PLACEMENT_3D('',#8487,#7112,#7113);
#6608=AXIS2_PLACEMENT_3D('',#8491,#7115,#7116);
#6609=AXIS2_PLACEMENT_3D('',#8492,#7117,#7118);
#6610=AXIS2_PLACEMENT_3D('',#8493,#7119,#7120);
#6611=AXIS2_PLACEMENT_3D('',#8497,#7123,#7124);
#6612=AXIS2_PLACEMENT_3D('',#8503,#7128,#7129);
#6613=AXIS2_PLACEMENT_3D('',#8512,#7134,#7135);
#6614=AXIS2_PLACEMENT_3D('',#8514,#7136,#7137);
#6615=AXIS2_PLACEMENT_3D('',#8516,#7138,#7139);
#6616=AXIS2_PLACEMENT_3D('',#8518,#7141,#7142);
#6617=AXIS2_PLACEMENT_3D('',#8519,#7143,#7144);
#6618=AXIS2_PLACEMENT_3D('',#8520,#7145,#7146);
#6619=AXIS2_PLACEMENT_3D('',#8521,#7147,#7148);
#6620=AXIS2_PLACEMENT_3D('',#8525,#7151,#7152);
#6621=AXIS2_PLACEMENT_3D('',#8533,#7157,#7158);
#6622=AXIS2_PLACEMENT_3D('',#8539,#7162,#7163);
#6623=AXIS2_PLACEMENT_3D('',#8545,#7167,#7168);
#6624=AXIS2_PLACEMENT_3D('',#8551,#7172,#7173);
#6625=AXIS2_PLACEMENT_3D('',#8553,#7174,#7175);
#6626=AXIS2_PLACEMENT_3D('',#8556,#7177,#7178);
#6627=AXIS2_PLACEMENT_3D('',#8557,#7179,#7180);
#6628=AXIS2_PLACEMENT_3D('',#8559,#7181,#7182);
#6629=AXIS2_PLACEMENT_3D('',#8562,#7184,#7185);
#6630=AXIS2_PLACEMENT_3D('',#8563,#7186,#7187);
#6631=AXIS2_PLACEMENT_3D('',#8567,#7189,#7190);
#6632=AXIS2_PLACEMENT_3D('',#8579,#7196,#7197);
#6633=AXIS2_PLACEMENT_3D('',#8584,#7200,#7201);
#6634=AXIS2_PLACEMENT_3D('',#8585,#7202,#7203);
#6635=AXIS2_PLACEMENT_3D('',#8587,#7204,#7205);
#6636=AXIS2_PLACEMENT_3D('',#8589,#7206,#7207);
#6637=AXIS2_PLACEMENT_3D('',#8590,#7208,#7209);
#6638=AXIS2_PLACEMENT_3D('',#8591,#7210,#7211);
#6639=AXIS2_PLACEMENT_3D('',#8594,#7212,#7213);
#6640=AXIS2_PLACEMENT_3D('',#8595,#7214,#7215);
#6641=AXIS2_PLACEMENT_3D('',#8597,#7217,#7218);
#6642=AXIS2_PLACEMENT_3D('',#8603,#7221,#7222);
#6643=AXIS2_PLACEMENT_3D('',#8615,#7228,#7229);
#6644=AXIS2_PLACEMENT_3D('',#8617,#7231,#7232);
#6645=AXIS2_PLACEMENT_3D('',#8618,#7233,#7234);
#6646=AXIS2_PLACEMENT_3D('',#8619,#7235,#7236);
#6647=AXIS2_PLACEMENT_3D('',#8622,#7239,#7240);
#6648=AXIS2_PLACEMENT_3D('',#8625,#7243,#7244);
#6649=AXIS2_PLACEMENT_3D('',#8627,#7246,#7247);
#6650=AXIS2_PLACEMENT_3D('',#8629,#7249,#7250);
#6651=AXIS2_PLACEMENT_3D('',#8630,#7251,#7252);
#6652=AXIS2_PLACEMENT_3D('',#8632,#7254,#7255);
#6653=AXIS2_PLACEMENT_3D('',#8633,#7256,#7257);
#6654=AXIS2_PLACEMENT_3D('',#8635,#7259,#7260);
#6655=AXIS2_PLACEMENT_3D('',#8637,#7262,#7263);
#7084=DIRECTION('axis',(0.,0.,1.));
#7085=DIRECTION('refdir',(1.,0.,0.));
#7086=DIRECTION('center_axis',(0.,0.,-1.));
#7087=DIRECTION('ref_axis',(1.,0.,0.));
#7088=DIRECTION('center_axis',(0.,0.,-1.));
#7089=DIRECTION('ref_axis',(1.,0.,0.));
#7090=DIRECTION('',(0.,0.,-1.));
#7091=DIRECTION('center_axis',(0.,0.,1.));
#7092=DIRECTION('ref_axis',(1.,0.,0.));
#7093=DIRECTION('center_axis',(0.,0.,-1.));
#7094=DIRECTION('ref_axis',(1.,0.,0.));
#7095=DIRECTION('center_axis',(0.,0.,-1.));
#7096=DIRECTION('ref_axis',(1.,0.,0.));
#7097=DIRECTION('',(0.,0.,-1.));
#7098=DIRECTION('center_axis',(0.,0.,1.));
#7099=DIRECTION('ref_axis',(1.,0.,0.));
#7100=DIRECTION('center_axis',(0.,0.,-1.));
#7101=DIRECTION('ref_axis',(1.,0.,0.));
#7102=DIRECTION('center_axis',(0.,0.,-1.));
#7103=DIRECTION('ref_axis',(1.,0.,0.));
#7104=DIRECTION('',(0.,0.,-1.));
#7105=DIRECTION('center_axis',(0.,0.,1.));
#7106=DIRECTION('ref_axis',(1.,0.,0.));
#7107=DIRECTION('center_axis',(0.852825510654705,0.52219598655729,2.98280813317006E-15));
#7108=DIRECTION('ref_axis',(-2.45173672180486E-15,-1.70798806265451E-15,
1.));
#7109=DIRECTION('',(0.52219598655729,-0.852825510654705,0.));
#7110=DIRECTION('',(-0.417756789245834,0.682260408523763,0.600000000000001));
#7111=DIRECTION('',(0.,0.,1.));
#7112=DIRECTION('center_axis',(0.,0.,-1.));
#7113=DIRECTION('ref_axis',(-0.52219598655729,-0.852825510654705,0.));
#7114=DIRECTION('',(0.417756789245831,0.682260408523765,0.600000000000001));
#7115=DIRECTION('center_axis',(0.,0.,1.));
#7116=DIRECTION('ref_axis',(-0.52219598655729,-0.852825510654705,0.));
#7117=DIRECTION('center_axis',(0.,0.,1.));
#7118=DIRECTION('ref_axis',(-0.52219598655729,-0.852825510654705,0.));
#7119=DIRECTION('center_axis',(0.852825510654705,-0.52219598655729,2.98280813317006E-15));
#7120=DIRECTION('ref_axis',(-2.63589301690668E-15,1.4072328089692E-15,1.));
#7121=DIRECTION('',(0.52219598655729,0.852825510654705,0.));
#7122=DIRECTION('',(0.,0.,1.));
#7123=DIRECTION('center_axis',(0.8,-0.6,0.));
#7124=DIRECTION('ref_axis',(0.6,0.8,0.));
#7125=DIRECTION('',(0.,0.,-1.));
#7126=DIRECTION('',(0.6,0.8,0.));
#7127=DIRECTION('',(-0.6,-0.8,0.));
#7128=DIRECTION('center_axis',(0.242535625036333,0.970142500145332,0.));
#7129=DIRECTION('ref_axis',(-0.970142500145332,0.242535625036333,0.));
#7130=DIRECTION('',(0.970142500145332,-0.242535625036333,0.));
#7131=DIRECTION('',(0.,0.,1.));
#7132=DIRECTION('',(-0.970142500145332,0.242535625036333,0.));
#7133=DIRECTION('',(0.,0.,1.));
#7134=DIRECTION('center_axis',(0.,0.,1.));
#7135=DIRECTION('ref_axis',(4.44089209850063E-15,1.,0.));
#7136=DIRECTION('center_axis',(0.,0.,1.));
#7137=DIRECTION('ref_axis',(4.44089209850063E-15,1.,0.));
#7138=DIRECTION('center_axis',(0.,0.,1.));
#7139=DIRECTION('ref_axis',(4.44089209850063E-15,1.,0.));
#7140=DIRECTION('',(0.,0.,1.));
#7141=DIRECTION('center_axis',(0.,0.,1.));
#7142=DIRECTION('ref_axis',(-0.0764170008251969,0.997075945946387,0.));
#7143=DIRECTION('center_axis',(0.,0.,1.));
#7144=DIRECTION('ref_axis',(-0.0764170008251969,0.997075945946387,0.));
#7145=DIRECTION('center_axis',(0.,0.,1.));
#7146=DIRECTION('ref_axis',(-0.0764170008251969,0.997075945946387,0.));
#7147=DIRECTION('center_axis',(0.,0.,1.));
#7148=DIRECTION('ref_axis',(1.,0.,0.));
#7149=DIRECTION('',(0.,-1.,0.));
#7150=DIRECTION('',(-1.,0.,0.));
#7151=DIRECTION('center_axis',(0.,1.,0.));
#7152=DIRECTION('ref_axis',(-1.,0.,0.));
#7153=DIRECTION('',(0.,0.,1.));
#7154=DIRECTION('',(-1.,0.,0.));
#7155=DIRECTION('',(0.,0.,1.));
#7156=DIRECTION('',(1.,0.,0.));
#7157=DIRECTION('center_axis',(-1.,0.,0.));
#7158=DIRECTION('ref_axis',(0.,-1.,0.));
#7159=DIRECTION('',(0.,1.,0.));
#7160=DIRECTION('',(0.,0.,1.));
#7161=DIRECTION('',(0.,-1.,0.));
#7162=DIRECTION('center_axis',(0.,-1.,0.));
#7163=DIRECTION('ref_axis',(1.,0.,0.));
#7164=DIRECTION('',(0.,0.,-1.));
#7165=DIRECTION('',(1.,0.,0.));
#7166=DIRECTION('',(-1.,0.,0.));
#7167=DIRECTION('center_axis',(1.,0.,0.));
#7168=DIRECTION('ref_axis',(0.,1.,0.));
#7169=DIRECTION('',(0.,0.,1.));
#7170=DIRECTION('',(0.,-1.,0.));
#7171=DIRECTION('',(0.,1.,0.));
#7172=DIRECTION('center_axis',(0.,0.,1.));
#7173=DIRECTION('ref_axis',(1.,0.,0.));
#7174=DIRECTION('center_axis',(0.,0.,1.));
#7175=DIRECTION('ref_axis',(1.,0.,0.));
#7176=DIRECTION('',(0.,0.,1.));
#7177=DIRECTION('center_axis',(0.,0.,1.));
#7178=DIRECTION('ref_axis',(1.,0.,0.));
#7179=DIRECTION('center_axis',(0.,0.,1.));
#7180=DIRECTION('ref_axis',(1.,0.,0.));
#7181=DIRECTION('center_axis',(0.,0.,1.));
#7182=DIRECTION('ref_axis',(1.,0.,0.));
#7183=DIRECTION('',(0.,0.,-1.));
#7184=DIRECTION('center_axis',(0.,0.,1.));
#7185=DIRECTION('ref_axis',(1.,0.,0.));
#7186=DIRECTION('center_axis',(0.,0.,1.));
#7187=DIRECTION('ref_axis',(1.,0.,0.));
#7188=DIRECTION('',(0.87524153543927,-0.483686111690123,0.));
#7189=DIRECTION('center_axis',(0.,0.,1.));
#7190=DIRECTION('ref_axis',(1.,0.,0.));
#7191=DIRECTION('',(0.87524153543927,-0.483686111690123,0.));
#7192=DIRECTION('',(1.,0.,0.));
#7193=DIRECTION('',(0.,1.,0.));
#7194=DIRECTION('',(-1.,0.,0.));
#7195=DIRECTION('',(-0.694594513699567,0.719401460617409,0.));
#7196=DIRECTION('center_axis',(0.,0.,1.));
#7197=DIRECTION('ref_axis',(1.,0.,0.));
#7198=DIRECTION('',(-0.694594513699567,0.719401460617409,0.));
#7199=DIRECTION('',(-0.447213595499958,-0.894427190999916,0.));
#7200=DIRECTION('center_axis',(0.,0.,1.));
#7201=DIRECTION('ref_axis',(-1.,0.,0.));
#7202=DIRECTION('center_axis',(0.,0.,1.));
#7203=DIRECTION('ref_axis',(1.,0.,0.));
#7204=DIRECTION('center_axis',(0.,0.,-1.));
#7205=DIRECTION('ref_axis',(-1.,2.01858731750028E-16,0.));
#7206=DIRECTION('center_axis',(0.,-1.,0.));
#7207=DIRECTION('ref_axis',(-1.,0.,0.));
#7208=DIRECTION('center_axis',(0.,0.,1.));
#7209=DIRECTION('ref_axis',(-1.,2.01858731750028E-16,0.));
#7210=DIRECTION('center_axis',(0.,0.,-1.));
#7211=DIRECTION('ref_axis',(1.,0.,0.));
#7212=DIRECTION('center_axis',(0.,0.,-1.));
#7213=DIRECTION('ref_axis',(-1.,0.,0.));
#7214=DIRECTION('center_axis',(0.,0.,-1.));
#7215=DIRECTION('ref_axis',(-1.,0.,0.));
#7216=DIRECTION('',(0.,0.,-1.));
#7217=DIRECTION('center_axis',(0.,0.,1.));
#7218=DIRECTION('ref_axis',(1.,0.,0.));
#7219=DIRECTION('',(-0.447213595499958,-0.894427190999916,0.));
#7220=DIRECTION('',(-0.694594513699567,0.719401460617409,0.));
#7221=DIRECTION('center_axis',(0.,0.,1.));
#7222=DIRECTION('ref_axis',(1.,0.,0.));
#7223=DIRECTION('',(-0.694594513699567,0.719401460617409,0.));
#7224=DIRECTION('',(-1.,0.,0.));
#7225=DIRECTION('',(0.,1.,0.));
#7226=DIRECTION('',(1.,0.,0.));
#7227=DIRECTION('',(0.87524153543927,-0.483686111690123,0.));
#7228=DIRECTION('center_axis',(0.,0.,1.));
#7229=DIRECTION('ref_axis',(1.,0.,0.));
#7230=DIRECTION('',(0.87524153543927,-0.483686111690123,0.));
#7231=DIRECTION('center_axis',(0.,0.,-1.));
#7232=DIRECTION('ref_axis',(-1.,0.,0.));
#7233=DIRECTION('center_axis',(0.,-1.,0.));
#7234=DIRECTION('ref_axis',(1.,0.,0.));
#7235=DIRECTION('center_axis',(0.,0.,1.));
#7236=DIRECTION('ref_axis',(1.,0.,0.));
#7237=DIRECTION('',(0.,0.,-1.));
#7238=DIRECTION('',(0.,0.,1.));
#7239=DIRECTION('center_axis',(0.,0.,1.));
#7240=DIRECTION('ref_axis',(-0.483686111690122,-0.87524153543927,0.));
#7241=DIRECTION('',(0.,0.,1.));
#7242=DIRECTION('',(0.,0.,-1.));
#7243=DIRECTION('center_axis',(-0.483686111690123,-0.87524153543927,0.));
#7244=DIRECTION('ref_axis',(0.87524153543927,-0.483686111690123,0.));
#7245=DIRECTION('',(0.,0.,1.));
#7246=DIRECTION('center_axis',(0.719401460617409,0.694594513699567,0.));
#7247=DIRECTION('ref_axis',(-0.694594513699567,0.719401460617409,0.));
#7248=DIRECTION('',(0.,0.,1.));
#7249=DIRECTION('center_axis',(-0.483686111690123,-0.87524153543927,0.));
#7250=DIRECTION('ref_axis',(0.87524153543927,-0.483686111690123,0.));
#7251=DIRECTION('center_axis',(-0.894427190999916,0.447213595499958,0.));
#7252=DIRECTION('ref_axis',(-0.447213595499958,-0.894427190999916,0.));
#7253=DIRECTION('',(0.,0.,1.));
#7254=DIRECTION('center_axis',(0.719401460617409,0.694594513699567,0.));
#7255=DIRECTION('ref_axis',(-0.694594513699567,0.719401460617409,0.));
#7256=DIRECTION('center_axis',(0.,1.,0.));
#7257=DIRECTION('ref_axis',(-1.,0.,0.));
#7258=DIRECTION('',(0.,0.,1.));
#7259=DIRECTION('center_axis',(1.,0.,0.));
#7260=DIRECTION('ref_axis',(0.,1.,0.));
#7261=DIRECTION('',(0.,0.,1.));
#7262=DIRECTION('center_axis',(0.,-1.,0.));
#7263=DIRECTION('ref_axis',(1.,0.,0.));
#8461=CARTESIAN_POINT('',(0.,0.,0.));
#8462=CARTESIAN_POINT('Origin',(6.,-2.5,0.3));
#8463=CARTESIAN_POINT('',(5.83,-2.5,0.6));
#8464=CARTESIAN_POINT('Origin',(6.,-2.5,0.6));
#8465=CARTESIAN_POINT('',(5.83,-2.5,0.));
#8466=CARTESIAN_POINT('',(5.83,-2.5,0.3));
#8467=CARTESIAN_POINT('Origin',(6.,-2.5,0.));
#8468=CARTESIAN_POINT('Origin',(14.,-2.5,0.3));
#8469=CARTESIAN_POINT('',(13.83,-2.5,0.6));
#8470=CARTESIAN_POINT('Origin',(14.,-2.5,0.6));
#8471=CARTESIAN_POINT('',(13.83,-2.5,0.));
#8472=CARTESIAN_POINT('',(13.83,-2.5,0.3));
#8473=CARTESIAN_POINT('Origin',(14.,-2.5,0.));
#8474=CARTESIAN_POINT('Origin',(0.,0.,0.3));
#8475=CARTESIAN_POINT('',(-0.41,5.02105187650415E-17,0.6));
#8476=CARTESIAN_POINT('Origin',(0.,0.,0.6));
#8477=CARTESIAN_POINT('',(-0.41,5.02105187650415E-17,0.));
#8478=CARTESIAN_POINT('',(-0.41,5.02105187650415E-17,0.3));
#8479=CARTESIAN_POINT('Origin',(0.,0.,0.));
#8480=CARTESIAN_POINT('Origin',(-2.29138429764753,-0.0507555356354263,0.175));
#8481=CARTESIAN_POINT('',(-2.40887839462292,0.141130204261882,0.3));
#8482=CARTESIAN_POINT('',(-2.2,-0.2,0.3));
#8483=CARTESIAN_POINT('',(-2.63798141173519,0.515290294708827,0.3));
#8484=CARTESIAN_POINT('',(-2.2,-0.2,0.));
#8485=CARTESIAN_POINT('',(-2.2,-0.199999999999998,1.9729463250961E-32));
#8486=CARTESIAN_POINT('',(-2.2,-0.2,0.));
#8487=CARTESIAN_POINT('Origin',(-4.5,3.55625,0.15));
#8488=CARTESIAN_POINT('',(-6.8,-0.2,0.));
#8489=CARTESIAN_POINT('',(-6.59112160537708,0.141130204261881,0.3));
#8490=CARTESIAN_POINT('',(-6.8,-0.200000000000001,1.9729463250961E-32));
#8491=CARTESIAN_POINT('Origin',(-4.5,3.55625,0.));
#8492=CARTESIAN_POINT('Origin',(-4.5,3.55625,0.3));
#8493=CARTESIAN_POINT('Origin',(-6.70861570235247,-0.0507555356354272,0.175));
#8494=CARTESIAN_POINT('',(-6.8,-0.2,0.3));
#8495=CARTESIAN_POINT('',(-6.3074808585895,0.604358706488338,0.3));
#8496=CARTESIAN_POINT('',(-6.8,-0.2,0.));
#8497=CARTESIAN_POINT('Origin',(-2.2,-0.2,0.));
#8498=CARTESIAN_POINT('',(-2.,0.0666666666666669,0.3));
#8499=CARTESIAN_POINT('',(-2.,0.0666666666666669,0.));
#8500=CARTESIAN_POINT('',(-2.,0.0666666666666667,0.));
#8501=CARTESIAN_POINT('',(-1.6,0.6,0.3));
#8502=CARTESIAN_POINT('',(-1.6,0.6,0.));
#8503=CARTESIAN_POINT('Origin',(-1.6,1.2,0.));
#8504=CARTESIAN_POINT('',(-2.4,1.4,0.));
#8505=CARTESIAN_POINT('',(-1.6,1.2,0.));
#8506=CARTESIAN_POINT('',(-2.4,1.4,0.));
#8507=CARTESIAN_POINT('',(-2.4,1.4,0.3));
#8508=CARTESIAN_POINT('',(-2.4,1.4,0.));
#8509=CARTESIAN_POINT('',(-1.6,1.2,0.3));
#8510=CARTESIAN_POINT('',(-2.4,1.4,0.3));
#8511=CARTESIAN_POINT('',(-1.6,1.2,0.));
#8512=CARTESIAN_POINT('Origin',(-6.8,1.38777878078145E-17,0.));
#8513=CARTESIAN_POINT('',(-6.8,0.200000000000001,0.));
#8514=CARTESIAN_POINT('Origin',(-6.8,1.38777878078145E-17,0.));
#8515=CARTESIAN_POINT('',(-6.8,0.200000000000002,0.3));
#8516=CARTESIAN_POINT('Origin',(-6.8,1.38777878078145E-17,0.3));
#8517=CARTESIAN_POINT('',(-6.8,0.200000000000001,0.));
#8518=CARTESIAN_POINT('Origin',(-1.47616279069767,-10.6540697674419,0.));
#8519=CARTESIAN_POINT('Origin',(-1.47616279069767,-10.6540697674419,0.));
#8520=CARTESIAN_POINT('Origin',(-1.47616279069767,-10.6540697674419,0.3));
#8521=CARTESIAN_POINT('Origin',(-4.3,0.275886703260749,0.3));
#8522=CARTESIAN_POINT('',(-2.,1.2,0.3));
#8523=CARTESIAN_POINT('',(-2.,0.737943351630374,0.3));
#8524=CARTESIAN_POINT('',(-2.75,1.2,0.3));
#8525=CARTESIAN_POINT('Origin',(-1.2,1.2,0.));
#8526=CARTESIAN_POINT('',(-2.,1.2,0.6));
#8527=CARTESIAN_POINT('',(-2.,1.2,0.));
#8528=CARTESIAN_POINT('',(-1.2,1.2,0.6));
#8529=CARTESIAN_POINT('',(-2.,1.2,0.6));
#8530=CARTESIAN_POINT('',(-1.2,1.2,0.));
#8531=CARTESIAN_POINT('',(-1.2,1.2,0.));
#8532=CARTESIAN_POINT('',(-2.,1.2,0.));
#8533=CARTESIAN_POINT('Origin',(-2.,1.2,0.));
#8534=CARTESIAN_POINT('',(-2.,0.,0.));
#8535=CARTESIAN_POINT('',(-2.,0.,0.));
#8536=CARTESIAN_POINT('',(-2.,0.,0.6));
#8537=CARTESIAN_POINT('',(-2.,0.,0.));
#8538=CARTESIAN_POINT('',(-2.,0.,0.6));
#8539=CARTESIAN_POINT('Origin',(-2.,0.,0.));
#8540=CARTESIAN_POINT('',(-1.4,0.,0.6));
#8541=CARTESIAN_POINT('',(-1.4,0.,0.));
#8542=CARTESIAN_POINT('',(-1.4,0.,0.));
#8543=CARTESIAN_POINT('',(-1.2,0.,0.6));
#8544=CARTESIAN_POINT('',(-1.2,0.,0.));
#8545=CARTESIAN_POINT('Origin',(-1.2,0.,0.));
#8546=CARTESIAN_POINT('',(-1.2,0.721110255092798,0.));
#8547=CARTESIAN_POINT('',(-1.2,0.721110255092798,0.6));
#8548=CARTESIAN_POINT('',(-1.2,0.721110255092798,0.));
#8549=CARTESIAN_POINT('',(-1.2,1.2,0.));
#8550=CARTESIAN_POINT('',(-1.2,1.2,0.6));
#8551=CARTESIAN_POINT('Origin',(0.,0.,0.));
#8552=CARTESIAN_POINT('',(0.533017816115691,-1.29456247732709,0.));
#8553=CARTESIAN_POINT('Origin',(0.,0.,0.));
#8554=CARTESIAN_POINT('',(0.533017816115691,-1.29456247732709,0.6));
#8555=CARTESIAN_POINT('',(0.533017816115691,-1.29456247732709,0.));
#8556=CARTESIAN_POINT('Origin',(0.,0.,0.6));
#8557=CARTESIAN_POINT('Origin',(0.,0.,0.));
#8558=CARTESIAN_POINT('',(0.993295878967653,0.986591757935306,0.6));
#8559=CARTESIAN_POINT('Origin',(0.,0.,0.6));
#8560=CARTESIAN_POINT('',(0.993295878967653,0.986591757935306,0.));
#8561=CARTESIAN_POINT('',(0.993295878967653,0.986591757935306,0.));
#8562=CARTESIAN_POINT('Origin',(0.,0.,0.));
#8563=CARTESIAN_POINT('Origin',(0.,0.,0.6));
#8564=CARTESIAN_POINT('',(0.549222100239177,-1.30351747644797,0.6));
#8565=CARTESIAN_POINT('',(0.,-1.,0.6));
#8566=CARTESIAN_POINT('',(3.51486278039743,-2.94242416811437,0.6));
#8567=CARTESIAN_POINT('Origin',(2.1,-2.,0.6));
#8568=CARTESIAN_POINT('',(3.8,-3.1,0.6));
#8569=CARTESIAN_POINT('',(0.,-1.,0.6));
#8570=CARTESIAN_POINT('',(15.2,-3.1,0.6));
#8571=CARTESIAN_POINT('',(3.8,-3.1,0.6));
#8572=CARTESIAN_POINT('',(15.2,-1.9,0.6));
#8573=CARTESIAN_POINT('',(15.2,-3.1,0.6));
#8574=CARTESIAN_POINT('',(3.8,-1.9,0.6));
#8575=CARTESIAN_POINT('',(15.2,-1.9,0.6));
#8576=CARTESIAN_POINT('',(3.79686161498349,-1.89674952980433,0.6));
#8577=CARTESIAN_POINT('',(3.8,-1.9,0.6));
#8578=CARTESIAN_POINT('',(2.26270761578574,-0.307804316349519,0.6));
#8579=CARTESIAN_POINT('Origin',(2.1,-2.,0.6));
#8580=CARTESIAN_POINT('',(1.,1.,0.6));
#8581=CARTESIAN_POINT('',(3.8,-1.9,0.6));
#8582=CARTESIAN_POINT('',(1.,1.,0.6));
#8583=CARTESIAN_POINT('',(3.3,-2.,0.6));
#8584=CARTESIAN_POINT('Origin',(2.1,-2.,0.6));
#8585=CARTESIAN_POINT('Origin',(2.1,-2.,0.1));
#8586=CARTESIAN_POINT('',(0.9,-2.,0.));
#8587=CARTESIAN_POINT('Origin',(2.1,-2.,0.));
#8588=CARTESIAN_POINT('',(1.,-2.,0.1));
#8589=CARTESIAN_POINT('Origin',(0.9,-2.,0.1));
#8590=CARTESIAN_POINT('Origin',(2.1,-2.,0.1));
#8591=CARTESIAN_POINT('Origin',(2.1,-2.,0.3));
#8592=CARTESIAN_POINT('',(3.2,-2.,0.5));
#8593=CARTESIAN_POINT('',(1.,-2.,0.5));
#8594=CARTESIAN_POINT('Origin',(2.1,-2.,0.5));
#8595=CARTESIAN_POINT('Origin',(2.1,-2.,0.5));
#8596=CARTESIAN_POINT('',(1.,-2.,0.3));
#8597=CARTESIAN_POINT('Origin',(0.,0.,0.));
#8598=CARTESIAN_POINT('',(1.,1.,0.));
#8599=CARTESIAN_POINT('',(1.,1.,0.));
#8600=CARTESIAN_POINT('',(2.26270761578574,-0.307804316349519,0.));
#8601=CARTESIAN_POINT('',(3.8,-1.9,0.));
#8602=CARTESIAN_POINT('',(3.79686161498349,-1.89674952980433,0.));
#8603=CARTESIAN_POINT('Origin',(2.1,-2.,0.));
#8604=CARTESIAN_POINT('',(3.8,-1.9,0.));
#8605=CARTESIAN_POINT('',(3.8,-1.9,0.));
#8606=CARTESIAN_POINT('',(15.2,-1.9,0.));
#8607=CARTESIAN_POINT('',(15.2,-1.9,0.));
#8608=CARTESIAN_POINT('',(15.2,-3.1,0.));
#8609=CARTESIAN_POINT('',(15.2,-3.1,0.));
#8610=CARTESIAN_POINT('',(3.8,-3.1,0.));
#8611=CARTESIAN_POINT('',(3.8,-3.1,0.));
#8612=CARTESIAN_POINT('',(3.51486278039743,-2.94242416811437,0.));
#8613=CARTESIAN_POINT('',(0.,-1.,0.));
#8614=CARTESIAN_POINT('',(0.549222100239177,-1.30351747644797,0.));
#8615=CARTESIAN_POINT('Origin',(2.1,-2.,0.));
#8616=CARTESIAN_POINT('',(0.,-1.,0.));
#8617=CARTESIAN_POINT('Origin',(2.1,-2.,0.5));
#8618=CARTESIAN_POINT('Origin',(3.3,-2.,0.5));
#8619=CARTESIAN_POINT('Origin',(2.1,-2.,0.));
#8620=CARTESIAN_POINT('',(2.26270761578574,-0.307804316349519,0.));
#8621=CARTESIAN_POINT('',(3.79686161498349,-1.89674952980433,0.));
#8622=CARTESIAN_POINT('Origin',(2.1,-2.,0.));
#8623=CARTESIAN_POINT('',(0.549222100239177,-1.30351747644797,0.));
#8624=CARTESIAN_POINT('',(3.51486278039743,-2.94242416811437,0.));
#8625=CARTESIAN_POINT('Origin',(0.,-1.,0.));
#8626=CARTESIAN_POINT('',(3.8,-3.1,0.));
#8627=CARTESIAN_POINT('Origin',(3.8,-1.9,0.));
#8628=CARTESIAN_POINT('',(3.8,-1.9,0.));
#8629=CARTESIAN_POINT('Origin',(0.,-1.,0.));
#8630=CARTESIAN_POINT('Origin',(1.,1.,0.));
#8631=CARTESIAN_POINT('',(1.,1.,0.));
#8632=CARTESIAN_POINT('Origin',(3.8,-1.9,0.));
#8633=CARTESIAN_POINT('Origin',(15.2,-1.9,0.));
#8634=CARTESIAN_POINT('',(15.2,-1.9,0.));
#8635=CARTESIAN_POINT('Origin',(15.2,-3.1,0.));
#8636=CARTESIAN_POINT('',(15.2,-3.1,0.));
#8637=CARTESIAN_POINT('Origin',(3.8,-3.1,0.));
#18331=UNCERTAINTY_MEASURE_WITH_UNIT(LENGTH_MEASURE(0.001),#18354,
'DISTANCE_ACCURACY_VALUE',
'Maximum model space distance between geometric entities at asserted c
onnectivities');
#18341=UNCERTAINTY_MEASURE_WITH_UNIT(LENGTH_MEASURE(0.001),#18354,
'DISTANCE_ACCURACY_VALUE',
'Maximum model space distance between geometric entities at asserted c
onnectivities');
#18343=(
GEOMETRIC_REPRESENTATION_CONTEXT(3)
GLOBAL_UNCERTAINTY_ASSIGNED_CONTEXT((#18331))
GLOBAL_UNIT_ASSIGNED_CONTEXT((#18354,#18356,#18357))
REPRESENTATION_CONTEXT('','3D')
);
#18353=(
GEOMETRIC_REPRESENTATION_CONTEXT(3)
GLOBAL_UNCERTAINTY_ASSIGNED_CONTEXT((#18341))
GLOBAL_UNIT_ASSIGNED_CONTEXT((#18354,#18356,#18357))
REPRESENTATION_CONTEXT('','3D')
);
#18354=(
LENGTH_UNIT()
NAMED_UNIT(*)
SI_UNIT(.CENTI.,.METRE.)
);
#18356=(
NAMED_UNIT(*)
PLANE_ANGLE_UNIT()
SI_UNIT($,.RADIAN.)
);
#18357=(
NAMED_UNIT(*)
SI_UNIT($,.STERADIAN.)
SOLID_ANGLE_UNIT()
);
#18359=SHAPE_DEFINITION_REPRESENTATION(#18370,#18397);
#18370=PRODUCT_DEFINITION_SHAPE('',$,#18409);
#18397=SHAPE_REPRESENTATION('',(#6596),#18343);
#18407=PRODUCT_DEFINITION_CONTEXT('part definition',#18442,'design');
#18409=PRODUCT_DEFINITION('Forged jaw and handle',
'Forged jaw and handle',#18420,#18407);
#18420=PRODUCT_DEFINITION_FORMATION('',$,#18445);
#18442=APPLICATION_CONTEXT(
'Core Data for Automotive Mechanical Design Process');
#18443=PRODUCT_CONTEXT('part definition',#18442,'mechanical');
#18445=PRODUCT('Forged jaw and handle','Forged jaw and handle',$,(#18443));
#18456=PRESENTATION_STYLE_ASSIGNMENT((#18464));
#18464=SURFACE_STYLE_USAGE(.BOTH.,#18472);
#18472=SURFACE_SIDE_STYLE('',(#18480));
#18480=SURFACE_STYLE_FILL_AREA(#18488);
#18488=FILL_AREA_STYLE('Tool steel gray',(#18496));
#18496=FILL_AREA_STYLE_COLOUR('Tool steel gray',#18504);
#18504=COLOUR_RGB('Tool steel gray',0.607843137254902,0.643137254901961,
0.698039215686274);
ENDSEC;
END-ISO-10303-21;
